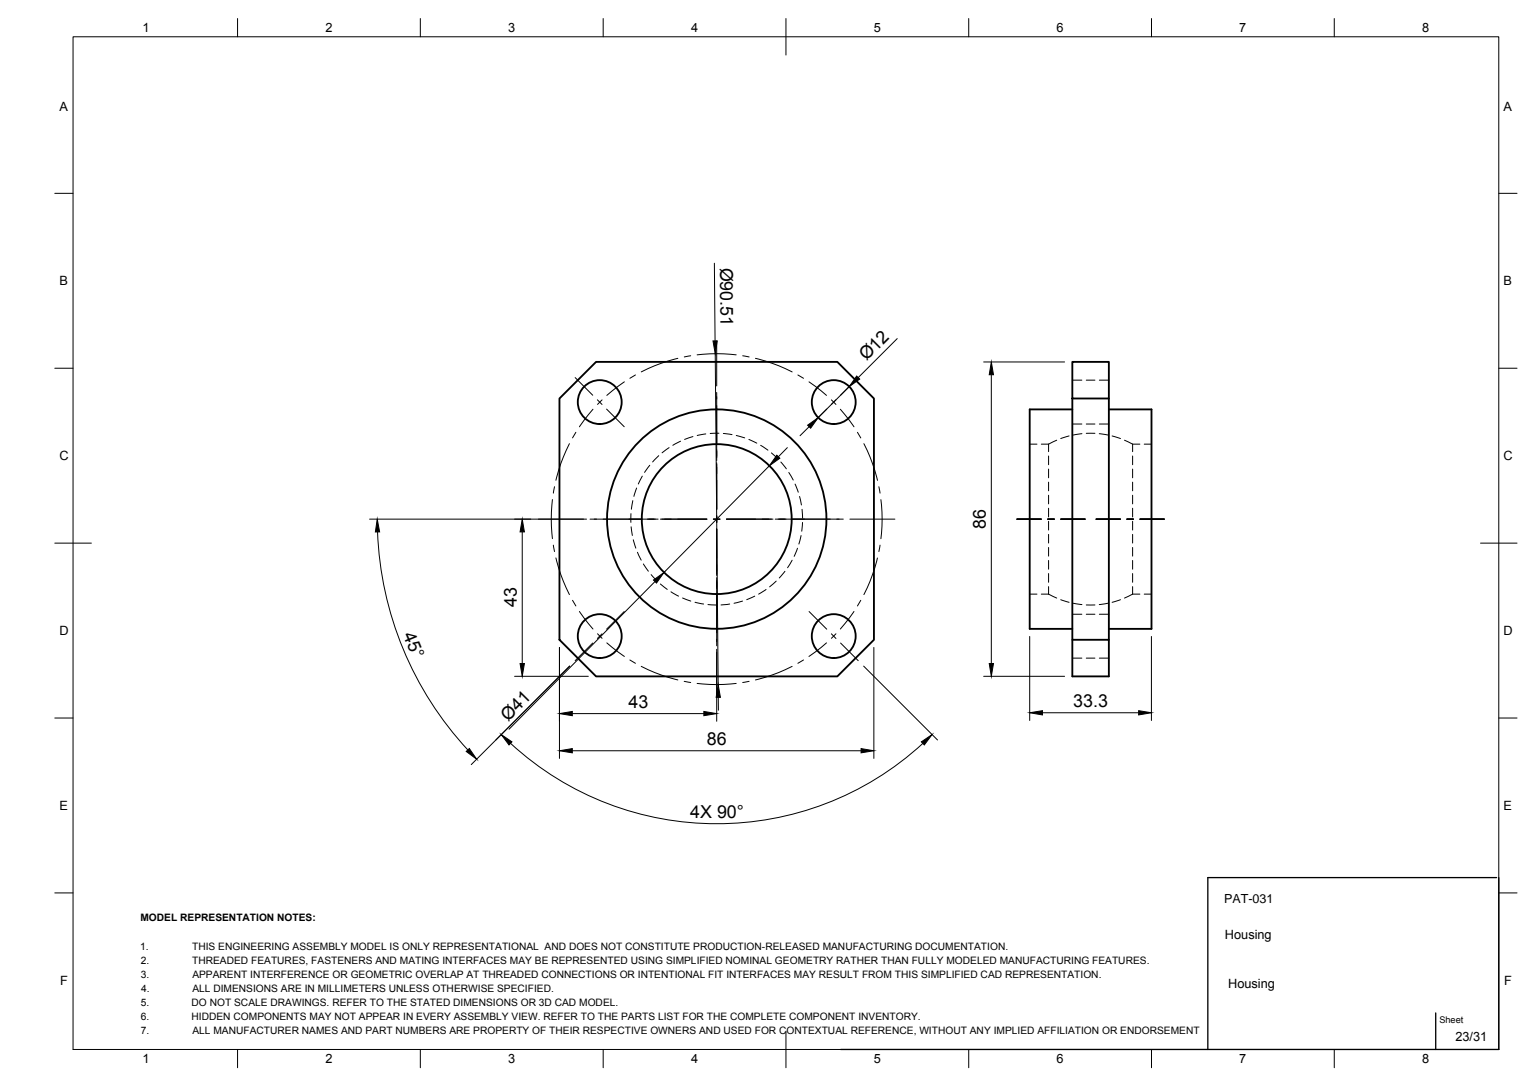
ISO-10303-21;
HEADER;
/* Generated by software containing ST-Developer
 * from STEP Tools, Inc. (www.steptools.com) 
 */

FILE_DESCRIPTION(
/* description */ ('Double-row support with tensioned shaft'),
/* implementation_level */ '2;1');

FILE_NAME(
/* name */ 'Housing.step',
/* time_stamp */ '2026-10-27T10:50:35-07:00',
/* author */ (''),
/* organization */ (''),
/* preprocessor_version */ 'ST-DEVELOPER v20.2',
/* originating_system */ 'Autodesk Translation Framework v15.17.0.0',
/* authorisation */ '');

FILE_SCHEMA (('AUTOMOTIVE_DESIGN { 1 0 10303 214 3 1 1 }'));
ENDSEC;

DATA;
#10=MECHANICAL_DESIGN_GEOMETRIC_PRESENTATION_REPRESENTATION('',(#498),#11559);
#391=SPHERICAL_SURFACE('',#7045,2.35);
#434=SHAPE_REPRESENTATION_RELATIONSHIP('SRR','None',#11743,#466);
#466=ADVANCED_BREP_SHAPE_REPRESENTATION('',(#529),#11545);
#498=STYLED_ITEM('',(#11946),#529);
#529=MANIFOLD_SOLID_BREP('Body1',#6345);
#615=FACE_BOUND('',#1534,.T.);
#616=FACE_BOUND('',#1535,.T.);
#617=FACE_BOUND('',#1539,.T.);
#618=FACE_BOUND('',#1541,.T.);
#619=FACE_BOUND('',#1555,.T.);
#620=FACE_BOUND('',#1556,.T.);
#621=FACE_BOUND('',#1557,.T.);
#622=FACE_BOUND('',#1558,.T.);
#623=FACE_BOUND('',#1559,.T.);
#624=FACE_BOUND('',#1561,.T.);
#625=FACE_BOUND('',#1562,.T.);
#626=FACE_BOUND('',#1563,.T.);
#627=FACE_BOUND('',#1564,.T.);
#628=FACE_BOUND('',#1565,.T.);
#822=PLANE('',#7053);
#823=PLANE('',#7054);
#824=PLANE('',#7067);
#825=PLANE('',#7068);
#826=PLANE('',#7069);
#827=PLANE('',#7070);
#828=PLANE('',#7071);
#829=PLANE('',#7072);
#830=PLANE('',#7073);
#831=PLANE('',#7074);
#832=PLANE('',#7075);
#833=PLANE('',#7076);
#1114=FACE_OUTER_BOUND('',#1531,.T.);
#1115=FACE_OUTER_BOUND('',#1532,.T.);
#1116=FACE_OUTER_BOUND('',#1533,.T.);
#1117=FACE_OUTER_BOUND('',#1536,.T.);
#1118=FACE_OUTER_BOUND('',#1537,.T.);
#1119=FACE_OUTER_BOUND('',#1538,.T.);
#1120=FACE_OUTER_BOUND('',#1540,.T.);
#1121=FACE_OUTER_BOUND('',#1542,.T.);
#1122=FACE_OUTER_BOUND('',#1543,.T.);
#1123=FACE_OUTER_BOUND('',#1544,.T.);
#1124=FACE_OUTER_BOUND('',#1545,.T.);
#1125=FACE_OUTER_BOUND('',#1546,.T.);
#1126=FACE_OUTER_BOUND('',#1547,.T.);
#1127=FACE_OUTER_BOUND('',#1548,.T.);
#1128=FACE_OUTER_BOUND('',#1549,.T.);
#1129=FACE_OUTER_BOUND('',#1550,.T.);
#1130=FACE_OUTER_BOUND('',#1551,.T.);
#1131=FACE_OUTER_BOUND('',#1552,.T.);
#1132=FACE_OUTER_BOUND('',#1553,.T.);
#1133=FACE_OUTER_BOUND('',#1554,.T.);
#1134=FACE_OUTER_BOUND('',#1560,.T.);
#1531=EDGE_LOOP('',(#5242,#5243,#5244,#5245));
#1532=EDGE_LOOP('',(#5246,#5247,#5248,#5249));
#1533=EDGE_LOOP('',(#5250,#5251));
#1534=EDGE_LOOP('',(#5252));
#1535=EDGE_LOOP('',(#5253));
#1536=EDGE_LOOP('',(#5254,#5255,#5256,#5257));
#1537=EDGE_LOOP('',(#5258,#5259,#5260,#5261));
#1538=EDGE_LOOP('',(#5262));
#1539=EDGE_LOOP('',(#5263));
#1540=EDGE_LOOP('',(#5264));
#1541=EDGE_LOOP('',(#5265));
#1542=EDGE_LOOP('',(#5266,#5267,#5268,#5269));
#1543=EDGE_LOOP('',(#5270,#5271,#5272,#5273));
#1544=EDGE_LOOP('',(#5274,#5275,#5276,#5277));
#1545=EDGE_LOOP('',(#5278,#5279,#5280,#5281));
#1546=EDGE_LOOP('',(#5282,#5283,#5284,#5285));
#1547=EDGE_LOOP('',(#5286,#5287,#5288,#5289));
#1548=EDGE_LOOP('',(#5290,#5291,#5292,#5293));
#1549=EDGE_LOOP('',(#5294,#5295,#5296,#5297));
#1550=EDGE_LOOP('',(#5298,#5299,#5300,#5301));
#1551=EDGE_LOOP('',(#5302,#5303,#5304,#5305));
#1552=EDGE_LOOP('',(#5306,#5307,#5308,#5309));
#1553=EDGE_LOOP('',(#5310,#5311,#5312,#5313));
#1554=EDGE_LOOP('',(#5314,#5315,#5316,#5317,#5318,#5319,#5320,#5321));
#1555=EDGE_LOOP('',(#5322));
#1556=EDGE_LOOP('',(#5323));
#1557=EDGE_LOOP('',(#5324));
#1558=EDGE_LOOP('',(#5325));
#1559=EDGE_LOOP('',(#5326));
#1560=EDGE_LOOP('',(#5327,#5328,#5329,#5330,#5331,#5332,#5333,#5334));
#1561=EDGE_LOOP('',(#5335));
#1562=EDGE_LOOP('',(#5336));
#1563=EDGE_LOOP('',(#5337));
#1564=EDGE_LOOP('',(#5338));
#1565=EDGE_LOOP('',(#5339));
#2092=LINE('',#10216,#2639);
#2093=LINE('',#10222,#2640);
#2094=LINE('',#10232,#2641);
#2095=LINE('',#10238,#2642);
#2096=LINE('',#10246,#2643);
#2097=LINE('',#10252,#2644);
#2098=LINE('',#10258,#2645);
#2099=LINE('',#10264,#2646);
#2100=LINE('',#10269,#2647);
#2101=LINE('',#10271,#2648);
#2102=LINE('',#10273,#2649);
#2103=LINE('',#10274,#2650);
#2104=LINE('',#10277,#2651);
#2105=LINE('',#10279,#2652);
#2106=LINE('',#10280,#2653);
#2107=LINE('',#10283,#2654);
#2108=LINE('',#10285,#2655);
#2109=LINE('',#10286,#2656);
#2110=LINE('',#10289,#2657);
#2111=LINE('',#10291,#2658);
#2112=LINE('',#10292,#2659);
#2113=LINE('',#10295,#2660);
#2114=LINE('',#10297,#2661);
#2115=LINE('',#10298,#2662);
#2116=LINE('',#10301,#2663);
#2117=LINE('',#10303,#2664);
#2118=LINE('',#10304,#2665);
#2119=LINE('',#10307,#2666);
#2120=LINE('',#10309,#2667);
#2121=LINE('',#10310,#2668);
#2122=LINE('',#10312,#2669);
#2123=LINE('',#10313,#2670);
#2639=VECTOR('',#8377,2.05);
#2640=VECTOR('',#8384,2.05);
#2641=VECTOR('',#8395,3.);
#2642=VECTOR('',#8402,3.);
#2643=VECTOR('',#8413,0.6);
#2644=VECTOR('',#8420,0.6);
#2645=VECTOR('',#8427,0.6);
#2646=VECTOR('',#8434,0.6);
#2647=VECTOR('',#8439,1.);
#2648=VECTOR('',#8440,1.);
#2649=VECTOR('',#8441,1.);
#2650=VECTOR('',#8442,1.);
#2651=VECTOR('',#8445,1.);
#2652=VECTOR('',#8446,1.);
#2653=VECTOR('',#8447,1.);
#2654=VECTOR('',#8450,1.);
#2655=VECTOR('',#8451,1.);
#2656=VECTOR('',#8452,1.);
#2657=VECTOR('',#8455,1.);
#2658=VECTOR('',#8456,1.);
#2659=VECTOR('',#8457,1.);
#2660=VECTOR('',#8460,1.);
#2661=VECTOR('',#8461,1.);
#2662=VECTOR('',#8462,1.);
#2663=VECTOR('',#8465,1.);
#2664=VECTOR('',#8466,1.);
#2665=VECTOR('',#8467,1.);
#2666=VECTOR('',#8470,1.);
#2667=VECTOR('',#8471,1.);
#2668=VECTOR('',#8472,1.);
#2669=VECTOR('',#8475,1.);
#2670=VECTOR('',#8476,1.);
#2940=CIRCLE('',#7040,2.05);
#2941=CIRCLE('',#7041,2.05);
#2942=CIRCLE('',#7043,2.05);
#2943=CIRCLE('',#7044,2.05);
#2944=CIRCLE('',#7046,2.35);
#2945=CIRCLE('',#7048,3.);
#2946=CIRCLE('',#7049,3.);
#2947=CIRCLE('',#7051,3.);
#2948=CIRCLE('',#7052,3.);
#2949=CIRCLE('',#7056,0.6);
#2950=CIRCLE('',#7057,0.6);
#2951=CIRCLE('',#7059,0.6);
#2952=CIRCLE('',#7060,0.6);
#2953=CIRCLE('',#7062,0.6);
#2954=CIRCLE('',#7063,0.6);
#2955=CIRCLE('',#7065,0.6);
#2956=CIRCLE('',#7066,0.6);
#3329=VERTEX_POINT('',#10213);
#3330=VERTEX_POINT('',#10215);
#3331=VERTEX_POINT('',#10219);
#3332=VERTEX_POINT('',#10221);
#3333=VERTEX_POINT('',#10225);
#3334=VERTEX_POINT('',#10226);
#3335=VERTEX_POINT('',#10229);
#3336=VERTEX_POINT('',#10231);
#3337=VERTEX_POINT('',#10235);
#3338=VERTEX_POINT('',#10237);
#3339=VERTEX_POINT('',#10243);
#3340=VERTEX_POINT('',#10245);
#3341=VERTEX_POINT('',#10249);
#3342=VERTEX_POINT('',#10251);
#3343=VERTEX_POINT('',#10255);
#3344=VERTEX_POINT('',#10257);
#3345=VERTEX_POINT('',#10261);
#3346=VERTEX_POINT('',#10263);
#3347=VERTEX_POINT('',#10267);
#3348=VERTEX_POINT('',#10268);
#3349=VERTEX_POINT('',#10270);
#3350=VERTEX_POINT('',#10272);
#3351=VERTEX_POINT('',#10276);
#3352=VERTEX_POINT('',#10278);
#3353=VERTEX_POINT('',#10282);
#3354=VERTEX_POINT('',#10284);
#3355=VERTEX_POINT('',#10288);
#3356=VERTEX_POINT('',#10290);
#3357=VERTEX_POINT('',#10294);
#3358=VERTEX_POINT('',#10296);
#3359=VERTEX_POINT('',#10300);
#3360=VERTEX_POINT('',#10302);
#3361=VERTEX_POINT('',#10306);
#3362=VERTEX_POINT('',#10308);
#4006=EDGE_CURVE('',#3329,#3329,#2940,.T.);
#4007=EDGE_CURVE('',#3329,#3330,#2092,.T.);
#4008=EDGE_CURVE('',#3330,#3330,#2941,.T.);
#4009=EDGE_CURVE('',#3331,#3331,#2942,.T.);
#4010=EDGE_CURVE('',#3331,#3332,#2093,.T.);
#4011=EDGE_CURVE('',#3332,#3332,#2943,.T.);
#4012=EDGE_CURVE('',#3333,#3334,#2944,.T.);
#4013=EDGE_CURVE('',#3335,#3335,#2945,.T.);
#4014=EDGE_CURVE('',#3335,#3336,#2094,.T.);
#4015=EDGE_CURVE('',#3336,#3336,#2946,.T.);
#4016=EDGE_CURVE('',#3337,#3337,#2947,.T.);
#4017=EDGE_CURVE('',#3337,#3338,#2095,.T.);
#4018=EDGE_CURVE('',#3338,#3338,#2948,.T.);
#4019=EDGE_CURVE('',#3339,#3339,#2949,.T.);
#4020=EDGE_CURVE('',#3339,#3340,#2096,.T.);
#4021=EDGE_CURVE('',#3340,#3340,#2950,.T.);
#4022=EDGE_CURVE('',#3341,#3341,#2951,.T.);
#4023=EDGE_CURVE('',#3341,#3342,#2097,.T.);
#4024=EDGE_CURVE('',#3342,#3342,#2952,.T.);
#4025=EDGE_CURVE('',#3343,#3343,#2953,.T.);
#4026=EDGE_CURVE('',#3343,#3344,#2098,.T.);
#4027=EDGE_CURVE('',#3344,#3344,#2954,.T.);
#4028=EDGE_CURVE('',#3345,#3345,#2955,.T.);
#4029=EDGE_CURVE('',#3345,#3346,#2099,.T.);
#4030=EDGE_CURVE('',#3346,#3346,#2956,.T.);
#4031=EDGE_CURVE('',#3347,#3348,#2100,.T.);
#4032=EDGE_CURVE('',#3348,#3349,#2101,.T.);
#4033=EDGE_CURVE('',#3350,#3349,#2102,.T.);
#4034=EDGE_CURVE('',#3347,#3350,#2103,.T.);
#4035=EDGE_CURVE('',#3351,#3347,#2104,.T.);
#4036=EDGE_CURVE('',#3352,#3350,#2105,.T.);
#4037=EDGE_CURVE('',#3351,#3352,#2106,.T.);
#4038=EDGE_CURVE('',#3353,#3351,#2107,.T.);
#4039=EDGE_CURVE('',#3354,#3352,#2108,.T.);
#4040=EDGE_CURVE('',#3353,#3354,#2109,.T.);
#4041=EDGE_CURVE('',#3355,#3353,#2110,.T.);
#4042=EDGE_CURVE('',#3356,#3354,#2111,.T.);
#4043=EDGE_CURVE('',#3355,#3356,#2112,.T.);
#4044=EDGE_CURVE('',#3357,#3355,#2113,.T.);
#4045=EDGE_CURVE('',#3358,#3356,#2114,.T.);
#4046=EDGE_CURVE('',#3357,#3358,#2115,.T.);
#4047=EDGE_CURVE('',#3359,#3357,#2116,.T.);
#4048=EDGE_CURVE('',#3360,#3358,#2117,.T.);
#4049=EDGE_CURVE('',#3359,#3360,#2118,.T.);
#4050=EDGE_CURVE('',#3361,#3359,#2119,.T.);
#4051=EDGE_CURVE('',#3362,#3360,#2120,.T.);
#4052=EDGE_CURVE('',#3361,#3362,#2121,.T.);
#4053=EDGE_CURVE('',#3348,#3361,#2122,.T.);
#4054=EDGE_CURVE('',#3349,#3362,#2123,.T.);
#5242=ORIENTED_EDGE('',*,*,#4006,.F.);
#5243=ORIENTED_EDGE('',*,*,#4007,.T.);
#5244=ORIENTED_EDGE('',*,*,#4008,.F.);
#5245=ORIENTED_EDGE('',*,*,#4007,.F.);
#5246=ORIENTED_EDGE('',*,*,#4009,.F.);
#5247=ORIENTED_EDGE('',*,*,#4010,.T.);
#5248=ORIENTED_EDGE('',*,*,#4011,.F.);
#5249=ORIENTED_EDGE('',*,*,#4010,.F.);
#5250=ORIENTED_EDGE('',*,*,#4012,.T.);
#5251=ORIENTED_EDGE('',*,*,#4012,.F.);
#5252=ORIENTED_EDGE('',*,*,#4009,.T.);
#5253=ORIENTED_EDGE('',*,*,#4008,.T.);
#5254=ORIENTED_EDGE('',*,*,#4013,.F.);
#5255=ORIENTED_EDGE('',*,*,#4014,.T.);
#5256=ORIENTED_EDGE('',*,*,#4015,.F.);
#5257=ORIENTED_EDGE('',*,*,#4014,.F.);
#5258=ORIENTED_EDGE('',*,*,#4016,.F.);
#5259=ORIENTED_EDGE('',*,*,#4017,.T.);
#5260=ORIENTED_EDGE('',*,*,#4018,.F.);
#5261=ORIENTED_EDGE('',*,*,#4017,.F.);
#5262=ORIENTED_EDGE('',*,*,#4015,.T.);
#5263=ORIENTED_EDGE('',*,*,#4006,.T.);
#5264=ORIENTED_EDGE('',*,*,#4016,.T.);
#5265=ORIENTED_EDGE('',*,*,#4011,.T.);
#5266=ORIENTED_EDGE('',*,*,#4019,.F.);
#5267=ORIENTED_EDGE('',*,*,#4020,.T.);
#5268=ORIENTED_EDGE('',*,*,#4021,.F.);
#5269=ORIENTED_EDGE('',*,*,#4020,.F.);
#5270=ORIENTED_EDGE('',*,*,#4022,.F.);
#5271=ORIENTED_EDGE('',*,*,#4023,.T.);
#5272=ORIENTED_EDGE('',*,*,#4024,.F.);
#5273=ORIENTED_EDGE('',*,*,#4023,.F.);
#5274=ORIENTED_EDGE('',*,*,#4025,.F.);
#5275=ORIENTED_EDGE('',*,*,#4026,.T.);
#5276=ORIENTED_EDGE('',*,*,#4027,.F.);
#5277=ORIENTED_EDGE('',*,*,#4026,.F.);
#5278=ORIENTED_EDGE('',*,*,#4028,.F.);
#5279=ORIENTED_EDGE('',*,*,#4029,.T.);
#5280=ORIENTED_EDGE('',*,*,#4030,.F.);
#5281=ORIENTED_EDGE('',*,*,#4029,.F.);
#5282=ORIENTED_EDGE('',*,*,#4031,.T.);
#5283=ORIENTED_EDGE('',*,*,#4032,.T.);
#5284=ORIENTED_EDGE('',*,*,#4033,.F.);
#5285=ORIENTED_EDGE('',*,*,#4034,.F.);
#5286=ORIENTED_EDGE('',*,*,#4035,.T.);
#5287=ORIENTED_EDGE('',*,*,#4034,.T.);
#5288=ORIENTED_EDGE('',*,*,#4036,.F.);
#5289=ORIENTED_EDGE('',*,*,#4037,.F.);
#5290=ORIENTED_EDGE('',*,*,#4038,.T.);
#5291=ORIENTED_EDGE('',*,*,#4037,.T.);
#5292=ORIENTED_EDGE('',*,*,#4039,.F.);
#5293=ORIENTED_EDGE('',*,*,#4040,.F.);
#5294=ORIENTED_EDGE('',*,*,#4041,.T.);
#5295=ORIENTED_EDGE('',*,*,#4040,.T.);
#5296=ORIENTED_EDGE('',*,*,#4042,.F.);
#5297=ORIENTED_EDGE('',*,*,#4043,.F.);
#5298=ORIENTED_EDGE('',*,*,#4044,.T.);
#5299=ORIENTED_EDGE('',*,*,#4043,.T.);
#5300=ORIENTED_EDGE('',*,*,#4045,.F.);
#5301=ORIENTED_EDGE('',*,*,#4046,.F.);
#5302=ORIENTED_EDGE('',*,*,#4047,.T.);
#5303=ORIENTED_EDGE('',*,*,#4046,.T.);
#5304=ORIENTED_EDGE('',*,*,#4048,.F.);
#5305=ORIENTED_EDGE('',*,*,#4049,.F.);
#5306=ORIENTED_EDGE('',*,*,#4050,.T.);
#5307=ORIENTED_EDGE('',*,*,#4049,.T.);
#5308=ORIENTED_EDGE('',*,*,#4051,.F.);
#5309=ORIENTED_EDGE('',*,*,#4052,.F.);
#5310=ORIENTED_EDGE('',*,*,#4053,.T.);
#5311=ORIENTED_EDGE('',*,*,#4052,.T.);
#5312=ORIENTED_EDGE('',*,*,#4054,.F.);
#5313=ORIENTED_EDGE('',*,*,#4032,.F.);
#5314=ORIENTED_EDGE('',*,*,#4054,.T.);
#5315=ORIENTED_EDGE('',*,*,#4051,.T.);
#5316=ORIENTED_EDGE('',*,*,#4048,.T.);
#5317=ORIENTED_EDGE('',*,*,#4045,.T.);
#5318=ORIENTED_EDGE('',*,*,#4042,.T.);
#5319=ORIENTED_EDGE('',*,*,#4039,.T.);
#5320=ORIENTED_EDGE('',*,*,#4036,.T.);
#5321=ORIENTED_EDGE('',*,*,#4033,.T.);
#5322=ORIENTED_EDGE('',*,*,#4018,.T.);
#5323=ORIENTED_EDGE('',*,*,#4021,.T.);
#5324=ORIENTED_EDGE('',*,*,#4024,.T.);
#5325=ORIENTED_EDGE('',*,*,#4027,.T.);
#5326=ORIENTED_EDGE('',*,*,#4030,.T.);
#5327=ORIENTED_EDGE('',*,*,#4053,.F.);
#5328=ORIENTED_EDGE('',*,*,#4031,.F.);
#5329=ORIENTED_EDGE('',*,*,#4035,.F.);
#5330=ORIENTED_EDGE('',*,*,#4038,.F.);
#5331=ORIENTED_EDGE('',*,*,#4041,.F.);
#5332=ORIENTED_EDGE('',*,*,#4044,.F.);
#5333=ORIENTED_EDGE('',*,*,#4047,.F.);
#5334=ORIENTED_EDGE('',*,*,#4050,.F.);
#5335=ORIENTED_EDGE('',*,*,#4013,.T.);
#5336=ORIENTED_EDGE('',*,*,#4019,.T.);
#5337=ORIENTED_EDGE('',*,*,#4022,.T.);
#5338=ORIENTED_EDGE('',*,*,#4025,.T.);
#5339=ORIENTED_EDGE('',*,*,#4028,.T.);
#5938=CYLINDRICAL_SURFACE('',#7039,2.05);
#5939=CYLINDRICAL_SURFACE('',#7042,2.05);
#5940=CYLINDRICAL_SURFACE('',#7047,3.);
#5941=CYLINDRICAL_SURFACE('',#7050,3.);
#5942=CYLINDRICAL_SURFACE('',#7055,0.6);
#5943=CYLINDRICAL_SURFACE('',#7058,0.6);
#5944=CYLINDRICAL_SURFACE('',#7061,0.6);
#5945=CYLINDRICAL_SURFACE('',#7064,0.6);
#6177=ADVANCED_FACE('',(#1114),#5938,.F.);
#6178=ADVANCED_FACE('',(#1115),#5939,.F.);
#6179=ADVANCED_FACE('',(#1116,#615,#616),#391,.F.);
#6180=ADVANCED_FACE('',(#1117),#5940,.T.);
#6181=ADVANCED_FACE('',(#1118),#5941,.T.);
#6182=ADVANCED_FACE('',(#1119,#617),#822,.F.);
#6183=ADVANCED_FACE('',(#1120,#618),#823,.T.);
#6184=ADVANCED_FACE('',(#1121),#5942,.F.);
#6185=ADVANCED_FACE('',(#1122),#5943,.F.);
#6186=ADVANCED_FACE('',(#1123),#5944,.F.);
#6187=ADVANCED_FACE('',(#1124),#5945,.F.);
#6188=ADVANCED_FACE('',(#1125),#824,.T.);
#6189=ADVANCED_FACE('',(#1126),#825,.T.);
#6190=ADVANCED_FACE('',(#1127),#826,.T.);
#6191=ADVANCED_FACE('',(#1128),#827,.T.);
#6192=ADVANCED_FACE('',(#1129),#828,.T.);
#6193=ADVANCED_FACE('',(#1130),#829,.T.);
#6194=ADVANCED_FACE('',(#1131),#830,.T.);
#6195=ADVANCED_FACE('',(#1132),#831,.T.);
#6196=ADVANCED_FACE('',(#1133,#619,#620,#621,#622,#623),#832,.T.);
#6197=ADVANCED_FACE('',(#1134,#624,#625,#626,#627,#628),#833,.F.);
#6345=CLOSED_SHELL('',(#6177,#6178,#6179,#6180,#6181,#6182,#6183,#6184,
#6185,#6186,#6187,#6188,#6189,#6190,#6191,#6192,#6193,#6194,#6195,#6196,
#6197));
#7038=AXIS2_PLACEMENT_3D('',#10211,#8371,#8372);
#7039=AXIS2_PLACEMENT_3D('',#10212,#8373,#8374);
#7040=AXIS2_PLACEMENT_3D('',#10214,#8375,#8376);
#7041=AXIS2_PLACEMENT_3D('',#10217,#8378,#8379);
#7042=AXIS2_PLACEMENT_3D('',#10218,#8380,#8381);
#7043=AXIS2_PLACEMENT_3D('',#10220,#8382,#8383);
#7044=AXIS2_PLACEMENT_3D('',#10223,#8385,#8386);
#7045=AXIS2_PLACEMENT_3D('',#10224,#8387,#8388);
#7046=AXIS2_PLACEMENT_3D('',#10227,#8389,#8390);
#7047=AXIS2_PLACEMENT_3D('',#10228,#8391,#8392);
#7048=AXIS2_PLACEMENT_3D('',#10230,#8393,#8394);
#7049=AXIS2_PLACEMENT_3D('',#10233,#8396,#8397);
#7050=AXIS2_PLACEMENT_3D('',#10234,#8398,#8399);
#7051=AXIS2_PLACEMENT_3D('',#10236,#8400,#8401);
#7052=AXIS2_PLACEMENT_3D('',#10239,#8403,#8404);
#7053=AXIS2_PLACEMENT_3D('',#10240,#8405,#8406);
#7054=AXIS2_PLACEMENT_3D('',#10241,#8407,#8408);
#7055=AXIS2_PLACEMENT_3D('',#10242,#8409,#8410);
#7056=AXIS2_PLACEMENT_3D('',#10244,#8411,#8412);
#7057=AXIS2_PLACEMENT_3D('',#10247,#8414,#8415);
#7058=AXIS2_PLACEMENT_3D('',#10248,#8416,#8417);
#7059=AXIS2_PLACEMENT_3D('',#10250,#8418,#8419);
#7060=AXIS2_PLACEMENT_3D('',#10253,#8421,#8422);
#7061=AXIS2_PLACEMENT_3D('',#10254,#8423,#8424);
#7062=AXIS2_PLACEMENT_3D('',#10256,#8425,#8426);
#7063=AXIS2_PLACEMENT_3D('',#10259,#8428,#8429);
#7064=AXIS2_PLACEMENT_3D('',#10260,#8430,#8431);
#7065=AXIS2_PLACEMENT_3D('',#10262,#8432,#8433);
#7066=AXIS2_PLACEMENT_3D('',#10265,#8435,#8436);
#7067=AXIS2_PLACEMENT_3D('',#10266,#8437,#8438);
#7068=AXIS2_PLACEMENT_3D('',#10275,#8443,#8444);
#7069=AXIS2_PLACEMENT_3D('',#10281,#8448,#8449);
#7070=AXIS2_PLACEMENT_3D('',#10287,#8453,#8454);
#7071=AXIS2_PLACEMENT_3D('',#10293,#8458,#8459);
#7072=AXIS2_PLACEMENT_3D('',#10299,#8463,#8464);
#7073=AXIS2_PLACEMENT_3D('',#10305,#8468,#8469);
#7074=AXIS2_PLACEMENT_3D('',#10311,#8473,#8474);
#7075=AXIS2_PLACEMENT_3D('',#10314,#8477,#8478);
#7076=AXIS2_PLACEMENT_3D('',#10315,#8479,#8480);
#8371=DIRECTION('axis',(0.,0.,1.));
#8372=DIRECTION('refdir',(1.,0.,0.));
#8373=DIRECTION('center_axis',(0.,1.,0.));
#8374=DIRECTION('ref_axis',(1.,0.,0.));
#8375=DIRECTION('center_axis',(0.,1.,0.));
#8376=DIRECTION('ref_axis',(1.,0.,0.));
#8377=DIRECTION('',(0.,1.,0.));
#8378=DIRECTION('center_axis',(0.,-1.,0.));
#8379=DIRECTION('ref_axis',(1.,0.,0.));
#8380=DIRECTION('center_axis',(0.,1.,0.));
#8381=DIRECTION('ref_axis',(1.,0.,0.));
#8382=DIRECTION('center_axis',(0.,1.,0.));
#8383=DIRECTION('ref_axis',(1.,0.,0.));
#8384=DIRECTION('',(0.,1.,0.));
#8385=DIRECTION('center_axis',(0.,-1.,0.));
#8386=DIRECTION('ref_axis',(1.,0.,0.));
#8387=DIRECTION('center_axis',(6.12323399573677E-17,0.,1.));
#8388=DIRECTION('ref_axis',(1.,0.,0.));
#8389=DIRECTION('center_axis',(-1.22464679914735E-16,1.,0.));
#8390=DIRECTION('ref_axis',(-1.,-1.22464679914735E-16,0.));
#8391=DIRECTION('center_axis',(0.,1.,0.));
#8392=DIRECTION('ref_axis',(1.,0.,0.));
#8393=DIRECTION('center_axis',(0.,1.,0.));
#8394=DIRECTION('ref_axis',(1.,0.,0.));
#8395=DIRECTION('',(0.,-1.,0.));
#8396=DIRECTION('center_axis',(0.,-1.,0.));
#8397=DIRECTION('ref_axis',(1.,0.,0.));
#8398=DIRECTION('center_axis',(0.,1.,0.));
#8399=DIRECTION('ref_axis',(1.,0.,0.));
#8400=DIRECTION('center_axis',(0.,1.,0.));
#8401=DIRECTION('ref_axis',(1.,0.,0.));
#8402=DIRECTION('',(0.,-1.,0.));
#8403=DIRECTION('center_axis',(0.,-1.,0.));
#8404=DIRECTION('ref_axis',(1.,0.,0.));
#8405=DIRECTION('center_axis',(0.,1.,0.));
#8406=DIRECTION('ref_axis',(1.,0.,0.));
#8407=DIRECTION('center_axis',(0.,1.,0.));
#8408=DIRECTION('ref_axis',(1.,0.,0.));
#8409=DIRECTION('center_axis',(0.,1.,0.));
#8410=DIRECTION('ref_axis',(1.,0.,0.));
#8411=DIRECTION('center_axis',(0.,1.,0.));
#8412=DIRECTION('ref_axis',(1.,0.,0.));
#8413=DIRECTION('',(0.,1.,0.));
#8414=DIRECTION('center_axis',(0.,-1.,0.));
#8415=DIRECTION('ref_axis',(1.,0.,0.));
#8416=DIRECTION('center_axis',(0.,1.,0.));
#8417=DIRECTION('ref_axis',(1.,0.,0.));
#8418=DIRECTION('center_axis',(0.,1.,0.));
#8419=DIRECTION('ref_axis',(1.,0.,0.));
#8420=DIRECTION('',(0.,1.,0.));
#8421=DIRECTION('center_axis',(0.,-1.,0.));
#8422=DIRECTION('ref_axis',(1.,0.,0.));
#8423=DIRECTION('center_axis',(0.,1.,0.));
#8424=DIRECTION('ref_axis',(1.,0.,0.));
#8425=DIRECTION('center_axis',(0.,1.,0.));
#8426=DIRECTION('ref_axis',(1.,0.,0.));
#8427=DIRECTION('',(0.,1.,0.));
#8428=DIRECTION('center_axis',(0.,-1.,0.));
#8429=DIRECTION('ref_axis',(1.,0.,0.));
#8430=DIRECTION('center_axis',(0.,1.,0.));
#8431=DIRECTION('ref_axis',(1.,0.,0.));
#8432=DIRECTION('center_axis',(0.,1.,0.));
#8433=DIRECTION('ref_axis',(1.,0.,0.));
#8434=DIRECTION('',(0.,1.,0.));
#8435=DIRECTION('center_axis',(0.,-1.,0.));
#8436=DIRECTION('ref_axis',(1.,0.,0.));
#8437=DIRECTION('center_axis',(-1.,0.,0.));
#8438=DIRECTION('ref_axis',(0.,0.,1.));
#8439=DIRECTION('',(0.,0.,1.));
#8440=DIRECTION('',(0.,1.,0.));
#8441=DIRECTION('',(0.,0.,1.));
#8442=DIRECTION('',(0.,1.,0.));
#8443=DIRECTION('center_axis',(-0.707106781186548,0.,-0.707106781186548));
#8444=DIRECTION('ref_axis',(-0.707106781186548,0.,0.707106781186548));
#8445=DIRECTION('',(-0.707106781186548,0.,0.707106781186548));
#8446=DIRECTION('',(-0.707106781186548,0.,0.707106781186548));
#8447=DIRECTION('',(0.,1.,0.));
#8448=DIRECTION('center_axis',(0.,0.,-1.));
#8449=DIRECTION('ref_axis',(-1.,0.,0.));
#8450=DIRECTION('',(-1.,0.,0.));
#8451=DIRECTION('',(-1.,0.,0.));
#8452=DIRECTION('',(0.,1.,0.));
#8453=DIRECTION('center_axis',(0.707106781186548,0.,-0.707106781186548));
#8454=DIRECTION('ref_axis',(-0.707106781186548,0.,-0.707106781186548));
#8455=DIRECTION('',(-0.707106781186548,0.,-0.707106781186548));
#8456=DIRECTION('',(-0.707106781186548,0.,-0.707106781186548));
#8457=DIRECTION('',(0.,1.,0.));
#8458=DIRECTION('center_axis',(1.,0.,0.));
#8459=DIRECTION('ref_axis',(0.,0.,-1.));
#8460=DIRECTION('',(0.,0.,-1.));
#8461=DIRECTION('',(0.,0.,-1.));
#8462=DIRECTION('',(0.,1.,0.));
#8463=DIRECTION('center_axis',(0.707106781186548,0.,0.707106781186548));
#8464=DIRECTION('ref_axis',(0.707106781186548,0.,-0.707106781186548));
#8465=DIRECTION('',(0.707106781186548,0.,-0.707106781186548));
#8466=DIRECTION('',(0.707106781186548,0.,-0.707106781186548));
#8467=DIRECTION('',(0.,1.,0.));
#8468=DIRECTION('center_axis',(0.,0.,1.));
#8469=DIRECTION('ref_axis',(1.,0.,0.));
#8470=DIRECTION('',(1.,0.,0.));
#8471=DIRECTION('',(1.,0.,0.));
#8472=DIRECTION('',(0.,1.,0.));
#8473=DIRECTION('center_axis',(-0.707106781186548,0.,0.707106781186548));
#8474=DIRECTION('ref_axis',(0.707106781186548,0.,0.707106781186548));
#8475=DIRECTION('',(0.707106781186548,0.,0.707106781186548));
#8476=DIRECTION('',(0.707106781186548,0.,0.707106781186548));
#8477=DIRECTION('center_axis',(0.,1.,0.));
#8478=DIRECTION('ref_axis',(0.,0.,1.));
#8479=DIRECTION('center_axis',(0.,1.,0.));
#8480=DIRECTION('ref_axis',(1.,0.,0.));
#10211=CARTESIAN_POINT('',(0.,0.,0.));
#10212=CARTESIAN_POINT('Origin',(0.,0.,0.));
#10213=CARTESIAN_POINT('',(-2.05,-1.665,2.51052593825207E-16));
#10214=CARTESIAN_POINT('Origin',(0.,-1.665,0.));
#10215=CARTESIAN_POINT('',(-2.05,-1.14891252930761,-2.51052593825207E-16));
#10216=CARTESIAN_POINT('',(-2.05,0.,2.51052593825207E-16));
#10217=CARTESIAN_POINT('Origin',(0.,-1.14891252930761,0.));
#10218=CARTESIAN_POINT('Origin',(0.,0.,0.));
#10219=CARTESIAN_POINT('',(-2.05,1.14891252930761,2.51052593825207E-16));
#10220=CARTESIAN_POINT('Origin',(0.,1.14891252930761,0.));
#10221=CARTESIAN_POINT('',(-2.05,1.665,-2.51052593825207E-16));
#10222=CARTESIAN_POINT('',(-2.05,0.,2.51052593825207E-16));
#10223=CARTESIAN_POINT('Origin',(0.,1.665,0.));
#10224=CARTESIAN_POINT('Origin',(0.,0.,0.));
#10225=CARTESIAN_POINT('',(-1.43895998899814E-16,-1.76221774462768E-32,
-2.35));
#10226=CARTESIAN_POINT('',(-1.43895998899814E-16,-1.76221774462768E-32,
2.35));
#10227=CARTESIAN_POINT('Origin',(0.,0.,0.));
#10228=CARTESIAN_POINT('Origin',(0.,0.,0.));
#10229=CARTESIAN_POINT('',(-3.,-0.5,3.67394039744206E-16));
#10230=CARTESIAN_POINT('Origin',(0.,-0.5,0.));
#10231=CARTESIAN_POINT('',(-3.,-1.665,3.67394039744206E-16));
#10232=CARTESIAN_POINT('',(-3.,0.,3.67394039744206E-16));
#10233=CARTESIAN_POINT('Origin',(0.,-1.665,0.));
#10234=CARTESIAN_POINT('Origin',(0.,0.,0.));
#10235=CARTESIAN_POINT('',(-3.,1.665,3.67394039744206E-16));
#10236=CARTESIAN_POINT('Origin',(0.,1.665,0.));
#10237=CARTESIAN_POINT('',(-3.,0.5,-3.67394039744206E-16));
#10238=CARTESIAN_POINT('',(-3.,0.,3.67394039744206E-16));
#10239=CARTESIAN_POINT('Origin',(0.,0.5,0.));
#10240=CARTESIAN_POINT('Origin',(0.,-1.665,0.));
#10241=CARTESIAN_POINT('Origin',(0.,1.665,0.));
#10242=CARTESIAN_POINT('Origin',(3.2,0.,3.2));
#10243=CARTESIAN_POINT('',(2.6,-0.5,3.2));
#10244=CARTESIAN_POINT('Origin',(3.2,-0.5,3.2));
#10245=CARTESIAN_POINT('',(2.6,0.5,3.2));
#10246=CARTESIAN_POINT('',(2.6,0.,3.2));
#10247=CARTESIAN_POINT('Origin',(3.2,0.5,3.2));
#10248=CARTESIAN_POINT('Origin',(-3.2,0.,-3.2));
#10249=CARTESIAN_POINT('',(-3.8,-0.5,-3.2));
#10250=CARTESIAN_POINT('Origin',(-3.2,-0.5,-3.2));
#10251=CARTESIAN_POINT('',(-3.8,0.5,-3.2));
#10252=CARTESIAN_POINT('',(-3.8,0.,-3.2));
#10253=CARTESIAN_POINT('Origin',(-3.2,0.5,-3.2));
#10254=CARTESIAN_POINT('Origin',(-3.2,0.,3.2));
#10255=CARTESIAN_POINT('',(-3.8,-0.5,3.2));
#10256=CARTESIAN_POINT('Origin',(-3.2,-0.5,3.2));
#10257=CARTESIAN_POINT('',(-3.8,0.5,3.2));
#10258=CARTESIAN_POINT('',(-3.8,0.,3.2));
#10259=CARTESIAN_POINT('Origin',(-3.2,0.5,3.2));
#10260=CARTESIAN_POINT('Origin',(3.2,0.,-3.2));
#10261=CARTESIAN_POINT('',(2.6,-0.5,-3.2));
#10262=CARTESIAN_POINT('Origin',(3.2,-0.5,-3.2));
#10263=CARTESIAN_POINT('',(2.6,0.5,-3.2));
#10264=CARTESIAN_POINT('',(2.6,0.,-3.2));
#10265=CARTESIAN_POINT('Origin',(3.2,0.5,-3.2));
#10266=CARTESIAN_POINT('Origin',(-4.3,-0.5,-3.3));
#10267=CARTESIAN_POINT('',(-4.3,-0.5,-3.3));
#10268=CARTESIAN_POINT('',(-4.3,-0.5,3.3));
#10269=CARTESIAN_POINT('',(-4.3,-0.5,-3.3));
#10270=CARTESIAN_POINT('',(-4.3,0.5,3.3));
#10271=CARTESIAN_POINT('',(-4.3,-0.5,3.3));
#10272=CARTESIAN_POINT('',(-4.3,0.5,-3.3));
#10273=CARTESIAN_POINT('',(-4.3,0.5,-3.3));
#10274=CARTESIAN_POINT('',(-4.3,-0.5,-3.3));
#10275=CARTESIAN_POINT('Origin',(-3.3,-0.5,-4.3));
#10276=CARTESIAN_POINT('',(-3.3,-0.5,-4.3));
#10277=CARTESIAN_POINT('',(-3.3,-0.5,-4.3));
#10278=CARTESIAN_POINT('',(-3.3,0.5,-4.3));
#10279=CARTESIAN_POINT('',(-3.3,0.5,-4.3));
#10280=CARTESIAN_POINT('',(-3.3,-0.5,-4.3));
#10281=CARTESIAN_POINT('Origin',(3.3,-0.5,-4.3));
#10282=CARTESIAN_POINT('',(3.3,-0.5,-4.3));
#10283=CARTESIAN_POINT('',(3.3,-0.5,-4.3));
#10284=CARTESIAN_POINT('',(3.3,0.5,-4.3));
#10285=CARTESIAN_POINT('',(3.3,0.5,-4.3));
#10286=CARTESIAN_POINT('',(3.3,-0.5,-4.3));
#10287=CARTESIAN_POINT('Origin',(4.3,-0.5,-3.3));
#10288=CARTESIAN_POINT('',(4.3,-0.5,-3.3));
#10289=CARTESIAN_POINT('',(4.3,-0.5,-3.3));
#10290=CARTESIAN_POINT('',(4.3,0.5,-3.3));
#10291=CARTESIAN_POINT('',(4.3,0.5,-3.3));
#10292=CARTESIAN_POINT('',(4.3,-0.5,-3.3));
#10293=CARTESIAN_POINT('Origin',(4.3,-0.5,3.3));
#10294=CARTESIAN_POINT('',(4.3,-0.5,3.3));
#10295=CARTESIAN_POINT('',(4.3,-0.5,3.3));
#10296=CARTESIAN_POINT('',(4.3,0.5,3.3));
#10297=CARTESIAN_POINT('',(4.3,0.5,3.3));
#10298=CARTESIAN_POINT('',(4.3,-0.5,3.3));
#10299=CARTESIAN_POINT('Origin',(3.3,-0.5,4.3));
#10300=CARTESIAN_POINT('',(3.3,-0.5,4.3));
#10301=CARTESIAN_POINT('',(3.3,-0.5,4.3));
#10302=CARTESIAN_POINT('',(3.3,0.5,4.3));
#10303=CARTESIAN_POINT('',(3.3,0.5,4.3));
#10304=CARTESIAN_POINT('',(3.3,-0.5,4.3));
#10305=CARTESIAN_POINT('Origin',(-3.3,-0.5,4.3));
#10306=CARTESIAN_POINT('',(-3.3,-0.5,4.3));
#10307=CARTESIAN_POINT('',(-3.3,-0.5,4.3));
#10308=CARTESIAN_POINT('',(-3.3,0.5,4.3));
#10309=CARTESIAN_POINT('',(-3.3,0.5,4.3));
#10310=CARTESIAN_POINT('',(-3.3,-0.5,4.3));
#10311=CARTESIAN_POINT('Origin',(-4.3,-0.5,3.3));
#10312=CARTESIAN_POINT('',(-4.3,-0.5,3.3));
#10313=CARTESIAN_POINT('',(-4.3,0.5,3.3));
#10314=CARTESIAN_POINT('Origin',(0.,0.5,0.));
#10315=CARTESIAN_POINT('Origin',(0.,-0.5,0.));
#11508=UNCERTAINTY_MEASURE_WITH_UNIT(LENGTH_MEASURE(0.001),#11560,
'DISTANCE_ACCURACY_VALUE',
'Maximum model space distance between geometric entities at asserted c
onnectivities');
#11522=UNCERTAINTY_MEASURE_WITH_UNIT(LENGTH_MEASURE(0.001),#11560,
'DISTANCE_ACCURACY_VALUE',
'Maximum model space distance between geometric entities at asserted c
onnectivities');
#11545=(
GEOMETRIC_REPRESENTATION_CONTEXT(3)
GLOBAL_UNCERTAINTY_ASSIGNED_CONTEXT((#11508))
GLOBAL_UNIT_ASSIGNED_CONTEXT((#11560,#11562,#11563))
REPRESENTATION_CONTEXT('','3D')
);
#11559=(
GEOMETRIC_REPRESENTATION_CONTEXT(3)
GLOBAL_UNCERTAINTY_ASSIGNED_CONTEXT((#11522))
GLOBAL_UNIT_ASSIGNED_CONTEXT((#11560,#11562,#11563))
REPRESENTATION_CONTEXT('','3D')
);
#11560=(
LENGTH_UNIT()
NAMED_UNIT(*)
SI_UNIT(.CENTI.,.METRE.)
);
#11562=(
NAMED_UNIT(*)
PLANE_ANGLE_UNIT()
SI_UNIT($,.RADIAN.)
);
#11563=(
NAMED_UNIT(*)
SI_UNIT($,.STERADIAN.)
SOLID_ANGLE_UNIT()
);
#11586=SHAPE_DEFINITION_REPRESENTATION(#11622,#11743);
#11622=PRODUCT_DEFINITION_SHAPE('',$,#11780);
#11743=SHAPE_REPRESENTATION('',(#7038),#11545);
#11757=PRODUCT_DEFINITION_CONTEXT('part definition',#11867,'design');
#11780=PRODUCT_DEFINITION('Housing','Housing',#11816,#11757);
#11816=PRODUCT_DEFINITION_FORMATION('',$,#11891);
#11867=APPLICATION_CONTEXT(
'Core Data for Automotive Mechanical Design Process');
#11868=PRODUCT_CONTEXT('part definition',#11867,'mechanical');
#11891=PRODUCT('Housing','Housing','Housing',(#11868));
#11940=COLOUR_RGB('Dark Blue',0.08,0.2,0.34);
#11941=FILL_AREA_STYLE_COLOUR('',#11940);
#11942=FILL_AREA_STYLE('',(#11941));
#11943=SURFACE_STYLE_FILL_AREA(#11942);
#11944=SURFACE_SIDE_STYLE('',(#11943));
#11945=SURFACE_STYLE_USAGE(.BOTH.,#11944);
#11946=PRESENTATION_STYLE_ASSIGNMENT((#11945));
ENDSEC;
END-ISO-10303-21;
